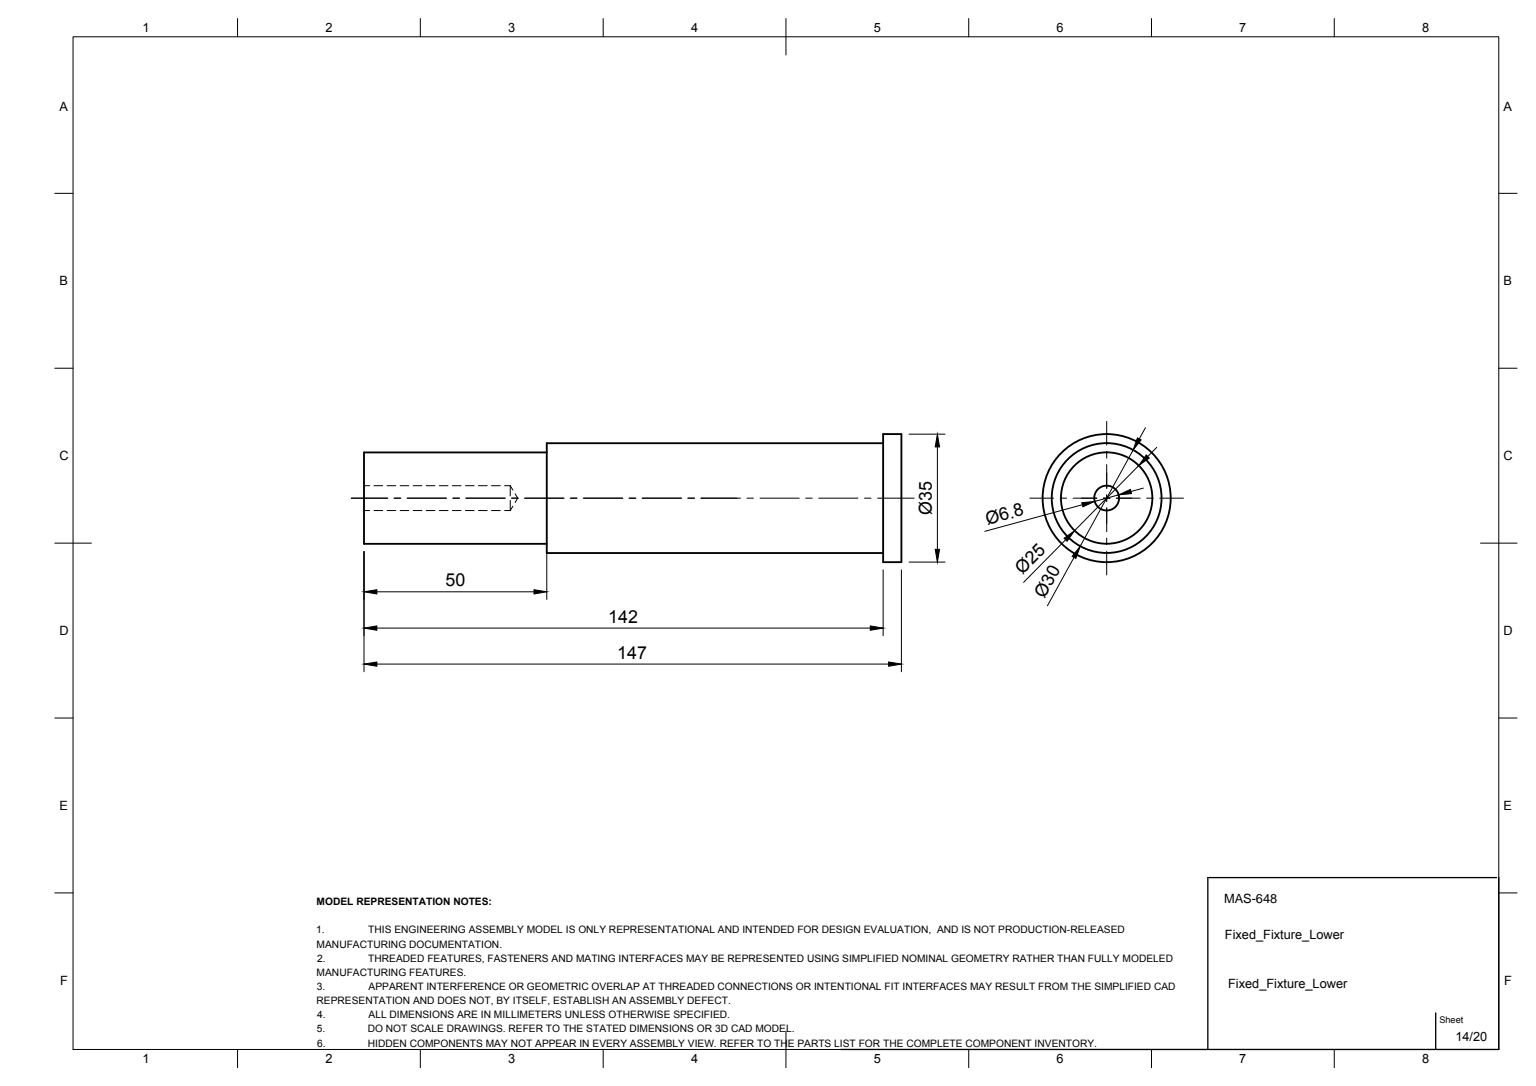
ISO-10303-21;
HEADER;
FILE_DESCRIPTION((''),'2;1');
FILE_NAME('Fixed_Fixture_Lower.step','2026-10-09T12:47:58-07:00',(''),(''),'','','');
FILE_SCHEMA (('AUTOMOTIVE_DESIGN { 1 0 10303 214 3 1 1 }'));
ENDSEC;
DATA;
#10=MECHANICAL_DESIGN_GEOMETRIC_PRESENTATION_REPRESENTATION('',(#317),#3475);
#33=CONICAL_SURFACE('',#2065,3.39999999999999,1.02974425867665) ;
#154=FACE_BOUND('',#522,.T.) ;
#155=FACE_BOUND('',#524,.T.) ;
#156=FACE_BOUND('',#526,.T.) ;
#190=CIRCLE('',#2063,3.39999999999999) ;
#191=CIRCLE('',#2064,3.39999999999999) ;
#192=CIRCLE('',#2067,12.5) ;
#193=CIRCLE('',#2068,12.5) ;
#194=CIRCLE('',#2070,15.) ;
#195=CIRCLE('',#2071,15.) ;
#196=CIRCLE('',#2073,17.5) ;
#197=CIRCLE('',#2074,17.5) ;
#269=CYLINDRICAL_SURFACE('',#2062,3.39999999999999) ;
#270=CYLINDRICAL_SURFACE('',#2066,12.5) ;
#271=CYLINDRICAL_SURFACE('',#2069,15.) ;
#272=CYLINDRICAL_SURFACE('',#2072,17.5) ;
#293=SHAPE_REPRESENTATION_RELATIONSHIP('SRR','None',#3548,#305) ;
#305=ADVANCED_BREP_SHAPE_REPRESENTATION('',(#329),#3468) ;
#317=STYLED_ITEM('',(#3628),#329) ;
#329=MANIFOLD_SOLID_BREP('Body1',#1831) ;
#388=FACE_OUTER_BOUND('',#515,.T.) ;
#389=FACE_OUTER_BOUND('',#516,.T.) ;
#390=FACE_OUTER_BOUND('',#517,.T.) ;
#391=FACE_OUTER_BOUND('',#518,.T.) ;
#392=FACE_OUTER_BOUND('',#519,.T.) ;
#393=FACE_OUTER_BOUND('',#520,.T.) ;
#394=FACE_OUTER_BOUND('',#521,.T.) ;
#395=FACE_OUTER_BOUND('',#523,.T.) ;
#396=FACE_OUTER_BOUND('',#525,.T.) ;
#515=EDGE_LOOP('',(#1414,#1415,#1416,#1417)) ;
#516=EDGE_LOOP('',(#1418,#1419,#1420)) ;
#517=EDGE_LOOP('',(#1421,#1422,#1423,#1424)) ;
#518=EDGE_LOOP('',(#1425,#1426,#1427,#1428)) ;
#519=EDGE_LOOP('',(#1429,#1430,#1431,#1432)) ;
#520=EDGE_LOOP('',(#1433)) ;
#521=EDGE_LOOP('',(#1434)) ;
#522=EDGE_LOOP('',(#1435)) ;
#523=EDGE_LOOP('',(#1436)) ;
#524=EDGE_LOOP('',(#1437)) ;
#525=EDGE_LOOP('',(#1438)) ;
#526=EDGE_LOOP('',(#1439)) ;
#669=LINE('',#3148,#788) ;
#670=LINE('',#3152,#789) ;
#671=LINE('',#3157,#790) ;
#672=LINE('',#3163,#791) ;
#673=LINE('',#3169,#792) ;
#788=VECTOR('',#2486,3.39999999999999) ;
#789=VECTOR('',#2491,3.39999999999999) ;
#790=VECTOR('',#2496,12.5) ;
#791=VECTOR('',#2503,15.) ;
#792=VECTOR('',#2510,17.5) ;
#898=VERTEX_POINT('',#3145) ;
#899=VERTEX_POINT('',#3147) ;
#900=VERTEX_POINT('',#3151) ;
#901=VERTEX_POINT('',#3154) ;
#902=VERTEX_POINT('',#3156) ;
#903=VERTEX_POINT('',#3160) ;
#904=VERTEX_POINT('',#3162) ;
#905=VERTEX_POINT('',#3166) ;
#906=VERTEX_POINT('',#3168) ;
#1079=EDGE_CURVE('',#898,#898,#190,.T.) ;
#1080=EDGE_CURVE('',#898,#899,#669,.T.) ;
#1081=EDGE_CURVE('',#899,#899,#191,.T.) ;
#1082=EDGE_CURVE('',#900,#898,#670,.T.) ;
#1083=EDGE_CURVE('',#901,#901,#192,.T.) ;
#1084=EDGE_CURVE('',#901,#902,#671,.T.) ;
#1085=EDGE_CURVE('',#902,#902,#193,.T.) ;
#1086=EDGE_CURVE('',#903,#903,#194,.T.) ;
#1087=EDGE_CURVE('',#903,#904,#672,.T.) ;
#1088=EDGE_CURVE('',#904,#904,#195,.T.) ;
#1089=EDGE_CURVE('',#905,#905,#196,.T.) ;
#1090=EDGE_CURVE('',#905,#906,#673,.T.) ;
#1091=EDGE_CURVE('',#906,#906,#197,.T.) ;
#1414=ORIENTED_EDGE('',*,*,#1079,.F.) ;
#1415=ORIENTED_EDGE('',*,*,#1080,.T.) ;
#1416=ORIENTED_EDGE('',*,*,#1081,.T.) ;
#1417=ORIENTED_EDGE('',*,*,#1080,.F.) ;
#1418=ORIENTED_EDGE('',*,*,#1082,.T.) ;
#1419=ORIENTED_EDGE('',*,*,#1079,.T.) ;
#1420=ORIENTED_EDGE('',*,*,#1082,.F.) ;
#1421=ORIENTED_EDGE('',*,*,#1083,.F.) ;
#1422=ORIENTED_EDGE('',*,*,#1084,.T.) ;
#1423=ORIENTED_EDGE('',*,*,#1085,.T.) ;
#1424=ORIENTED_EDGE('',*,*,#1084,.F.) ;
#1425=ORIENTED_EDGE('',*,*,#1086,.F.) ;
#1426=ORIENTED_EDGE('',*,*,#1087,.T.) ;
#1427=ORIENTED_EDGE('',*,*,#1088,.T.) ;
#1428=ORIENTED_EDGE('',*,*,#1087,.F.) ;
#1429=ORIENTED_EDGE('',*,*,#1089,.F.) ;
#1430=ORIENTED_EDGE('',*,*,#1090,.T.) ;
#1431=ORIENTED_EDGE('',*,*,#1091,.T.) ;
#1432=ORIENTED_EDGE('',*,*,#1090,.F.) ;
#1433=ORIENTED_EDGE('',*,*,#1091,.F.) ;
#1434=ORIENTED_EDGE('',*,*,#1089,.T.) ;
#1435=ORIENTED_EDGE('',*,*,#1088,.F.) ;
#1436=ORIENTED_EDGE('',*,*,#1086,.T.) ;
#1437=ORIENTED_EDGE('',*,*,#1085,.F.) ;
#1438=ORIENTED_EDGE('',*,*,#1083,.T.) ;
#1439=ORIENTED_EDGE('',*,*,#1081,.F.) ;
#1683=PLANE('',#2075) ;
#1684=PLANE('',#2076) ;
#1685=PLANE('',#2077) ;
#1686=PLANE('',#2078) ;
#1764=ADVANCED_FACE('',(#388),#269,.F.) ;
#1765=ADVANCED_FACE('',(#389),#33,.F.) ;
#1766=ADVANCED_FACE('',(#390),#270,.T.) ;
#1767=ADVANCED_FACE('',(#391),#271,.T.) ;
#1768=ADVANCED_FACE('',(#392),#272,.T.) ;
#1769=ADVANCED_FACE('',(#393),#1683,.T.) ;
#1770=ADVANCED_FACE('',(#394,#154),#1684,.T.) ;
#1771=ADVANCED_FACE('',(#395,#155),#1685,.T.) ;
#1772=ADVANCED_FACE('',(#396,#156),#1686,.T.) ;
#1831=CLOSED_SHELL('',(#1764,#1765,#1766,#1767,#1768,#1769,#1770,#1771,
#1772)) ;
#2061=AXIS2_PLACEMENT_3D('',#3143,#2480,#2481) ;
#2062=AXIS2_PLACEMENT_3D('',#3144,#2482,#2483) ;
#2063=AXIS2_PLACEMENT_3D('',#3146,#2484,#2485) ;
#2064=AXIS2_PLACEMENT_3D('',#3149,#2487,#2488) ;
#2065=AXIS2_PLACEMENT_3D('',#3150,#2489,#2490) ;
#2066=AXIS2_PLACEMENT_3D('',#3153,#2492,#2493) ;
#2067=AXIS2_PLACEMENT_3D('',#3155,#2494,#2495) ;
#2068=AXIS2_PLACEMENT_3D('',#3158,#2497,#2498) ;
#2069=AXIS2_PLACEMENT_3D('',#3159,#2499,#2500) ;
#2070=AXIS2_PLACEMENT_3D('',#3161,#2501,#2502) ;
#2071=AXIS2_PLACEMENT_3D('',#3164,#2504,#2505) ;
#2072=AXIS2_PLACEMENT_3D('',#3165,#2506,#2507) ;
#2073=AXIS2_PLACEMENT_3D('',#3167,#2508,#2509) ;
#2074=AXIS2_PLACEMENT_3D('',#3170,#2511,#2512) ;
#2075=AXIS2_PLACEMENT_3D('',#3171,#2513,#2514) ;
#2076=AXIS2_PLACEMENT_3D('',#3172,#2515,#2516) ;
#2077=AXIS2_PLACEMENT_3D('',#3173,#2517,#2518) ;
#2078=AXIS2_PLACEMENT_3D('',#3174,#2519,#2520) ;
#2480=DIRECTION('axis',(0.,0.,1.)) ;
#2481=DIRECTION('refdir',(1.,0.,0.)) ;
#2482=DIRECTION('center_axis',(1.,0.,0.)) ;
#2483=DIRECTION('ref_axis',(0.,0.,-1.)) ;
#2484=DIRECTION('center_axis',(1.,0.,0.)) ;
#2485=DIRECTION('ref_axis',(0.,0.,-1.)) ;
#2486=DIRECTION('',(1.,0.,0.)) ;
#2487=DIRECTION('center_axis',(1.,0.,0.)) ;
#2488=DIRECTION('ref_axis',(0.,0.,-1.)) ;
#2489=DIRECTION('center_axis',(1.,0.,0.)) ;
#2490=DIRECTION('ref_axis',(0.,0.,-1.)) ;
#2491=DIRECTION('',(0.515038074910058,-1.04972719113862E-16,0.85716730070211)) ;
#2492=DIRECTION('center_axis',(1.,-1.18008399726313E-17,0.)) ;
#2493=DIRECTION('ref_axis',(1.18008399726313E-17,1.,0.)) ;
#2494=DIRECTION('center_axis',(1.,-1.18008399726313E-17,0.)) ;
#2495=DIRECTION('ref_axis',(1.18008399726313E-17,1.,0.)) ;
#2496=DIRECTION('',(-1.,1.18008399726313E-17,0.)) ;
#2497=DIRECTION('center_axis',(1.,-1.18008399726313E-17,0.)) ;
#2498=DIRECTION('ref_axis',(1.18008399726313E-17,1.,0.)) ;
#2499=DIRECTION('center_axis',(1.,-1.18008399726313E-17,0.)) ;
#2500=DIRECTION('ref_axis',(1.18008399726313E-17,1.,0.)) ;
#2501=DIRECTION('center_axis',(1.,-1.18008399726313E-17,0.)) ;
#2502=DIRECTION('ref_axis',(1.18008399726313E-17,1.,0.)) ;
#2503=DIRECTION('',(-1.,1.18008399726313E-17,0.)) ;
#2504=DIRECTION('center_axis',(1.,-1.18008399726313E-17,0.)) ;
#2505=DIRECTION('ref_axis',(1.18008399726313E-17,1.,0.)) ;
#2506=DIRECTION('center_axis',(1.,-1.18008399726313E-17,0.)) ;
#2507=DIRECTION('ref_axis',(1.18008399726313E-17,1.,0.)) ;
#2508=DIRECTION('center_axis',(1.,-1.18008399726313E-17,0.)) ;
#2509=DIRECTION('ref_axis',(1.18008399726313E-17,1.,0.)) ;
#2510=DIRECTION('',(-1.,1.18008399726313E-17,0.)) ;
#2511=DIRECTION('center_axis',(1.,-1.18008399726313E-17,0.)) ;
#2512=DIRECTION('ref_axis',(1.18008399726313E-17,1.,0.)) ;
#2513=DIRECTION('center_axis',(-1.,1.18008399726313E-17,0.)) ;
#2514=DIRECTION('ref_axis',(-1.18008399726313E-17,-1.,0.)) ;
#2515=DIRECTION('center_axis',(1.,-1.18008399726313E-17,0.)) ;
#2516=DIRECTION('ref_axis',(1.18008399726313E-17,1.,0.)) ;
#2517=DIRECTION('center_axis',(1.,-1.18008399726313E-17,0.)) ;
#2518=DIRECTION('ref_axis',(1.18008399726313E-17,1.,0.)) ;
#2519=DIRECTION('center_axis',(1.,-1.18008399726313E-17,0.)) ;
#2520=DIRECTION('ref_axis',(1.18008399726313E-17,1.,0.)) ;
#3143=CARTESIAN_POINT('',(0.,0.,0.)) ;
#3144=CARTESIAN_POINT('Origin',(147.,-1.73472347597681E-15,0.)) ;
#3145=CARTESIAN_POINT('',(107.,-2.15110338768691E-15,3.39999999999999)) ;
#3146=CARTESIAN_POINT('Origin',(107.,-1.73472347597681E-15,0.)) ;
#3147=CARTESIAN_POINT('',(147.,-2.15110338768691E-15,3.39999999999999)) ;
#3148=CARTESIAN_POINT('',(147.,-2.15110338768691E-15,3.39999999999999)) ;
#3149=CARTESIAN_POINT('Origin',(147.,-1.73472347597681E-15,0.)) ;
#3150=CARTESIAN_POINT('Origin',(107.,-1.73472347597681E-15,0.)) ;
#3151=CARTESIAN_POINT('',(104.957073895306,-1.35382008469159E-14,0.)) ;
#3152=CARTESIAN_POINT('',(107.,-2.15110338768691E-15,3.39999999999999)) ;
#3153=CARTESIAN_POINT('Origin',(147.,-1.73472347597681E-15,0.)) ;
#3154=CARTESIAN_POINT('',(147.,-12.5,-1.53080849893419E-15)) ;
#3155=CARTESIAN_POINT('Origin',(147.,-1.73472347597681E-15,0.)) ;
#3156=CARTESIAN_POINT('',(97.,-12.5,-1.53080849893419E-15)) ;
#3157=CARTESIAN_POINT('',(147.,-12.5,-1.53080849893419E-15)) ;
#3158=CARTESIAN_POINT('Origin',(97.,-1.14468147734524E-15,0.)) ;
#3159=CARTESIAN_POINT('Origin',(147.,-1.73472347597681E-15,0.)) ;
#3160=CARTESIAN_POINT('',(97.,-15.,-1.83697019872103E-15)) ;
#3161=CARTESIAN_POINT('Origin',(97.,-1.14468147734524E-15,0.)) ;
#3162=CARTESIAN_POINT('',(5.,-15.,-1.83697019872103E-15)) ;
#3163=CARTESIAN_POINT('',(147.,-15.,-1.83697019872103E-15)) ;
#3164=CARTESIAN_POINT('Origin',(5.,-5.90041998631564E-17,0.)) ;
#3165=CARTESIAN_POINT('Origin',(147.,-1.73472347597681E-15,0.)) ;
#3166=CARTESIAN_POINT('',(5.,-17.5,-2.14313189850787E-15)) ;
#3167=CARTESIAN_POINT('Origin',(5.,-5.90041998631564E-17,0.)) ;
#3168=CARTESIAN_POINT('',(0.,-17.5,-2.14313189850787E-15)) ;
#3169=CARTESIAN_POINT('',(147.,-17.5,-2.14313189850787E-15)) ;
#3170=CARTESIAN_POINT('Origin',(0.,3.85185988877447E-31,0.)) ;
#3171=CARTESIAN_POINT('Origin',(-1.03257349760524E-16,1.21852346052197E-33,
0.)) ;
#3172=CARTESIAN_POINT('Origin',(5.,17.5,0.)) ;
#3173=CARTESIAN_POINT('Origin',(97.,15.,0.)) ;
#3174=CARTESIAN_POINT('Origin',(147.,12.5,0.)) ;
#3450=UNCERTAINTY_MEASURE_WITH_UNIT(LENGTH_MEASURE(0.01),#3476,
'DISTANCE_ACCURACY_VALUE',
'Maximum model space distance between geometric entities at asserted c
onnectivities') ;
#3457=UNCERTAINTY_MEASURE_WITH_UNIT(LENGTH_MEASURE(0.01),#3476,
'DISTANCE_ACCURACY_VALUE',
'Maximum model space distance between geometric entities at asserted c
onnectivities') ;
#3468=(
GEOMETRIC_REPRESENTATION_CONTEXT(3)
GLOBAL_UNCERTAINTY_ASSIGNED_CONTEXT((#3450))
GLOBAL_UNIT_ASSIGNED_CONTEXT((#3476,#3478,#3479))
REPRESENTATION_CONTEXT('','3D')
) ;
#3475=(
GEOMETRIC_REPRESENTATION_CONTEXT(3)
GLOBAL_UNCERTAINTY_ASSIGNED_CONTEXT((#3457))
GLOBAL_UNIT_ASSIGNED_CONTEXT((#3476,#3478,#3479))
REPRESENTATION_CONTEXT('','3D')
) ;
#3476=(
LENGTH_UNIT()
NAMED_UNIT(*)
SI_UNIT(.MILLI.,.METRE.)
) ;
#3478=(
NAMED_UNIT(*)
PLANE_ANGLE_UNIT()
SI_UNIT($,.RADIAN.)
) ;
#3479=(
NAMED_UNIT(*)
SI_UNIT($,.STERADIAN.)
SOLID_ANGLE_UNIT()
) ;
#3490=SHAPE_DEFINITION_REPRESENTATION(#3511,#3548) ;
#3511=PRODUCT_DEFINITION_SHAPE('',$,#3566) ;
#3548=SHAPE_REPRESENTATION('',(#2061),#3468) ;
#3555=PRODUCT_DEFINITION_CONTEXT('part definition',#3608,'design') ;
#3566=PRODUCT_DEFINITION(
'Fixed_Fixture_Lower',
'Fixed_Fixture_Lower',#3583,#3555) ;
#3583=PRODUCT_DEFINITION_FORMATION('',$,#3620) ;
#3608=APPLICATION_CONTEXT(
'Core Data for Automotive Mechanical Design Process') ;
#3609=PRODUCT_CONTEXT('part definition',#3608,'mechanical') ;
#3620=PRODUCT('Fixed_Fixture_Lower',
'Fixed_Fixture_Lower',$,(#3609)) ;
#3628=PRESENTATION_STYLE_ASSIGNMENT((#3630)) ;
#3630=SURFACE_STYLE_USAGE(.BOTH.,#3632) ;
#3632=SURFACE_SIDE_STYLE('',(#3634)) ;
#3634=SURFACE_STYLE_FILL_AREA(#3636) ;
#3636=FILL_AREA_STYLE('Opaque(202,209,238)',(#3638)) ;
#3638=FILL_AREA_STYLE_COLOUR('Opaque(202,209,238)',#3640) ;
#3640=COLOUR_RGB('Opaque(202,209,238)', 0.09019608, 0.27058824, 0.51372549) ;
ENDSEC;
END-ISO-10303-21;
